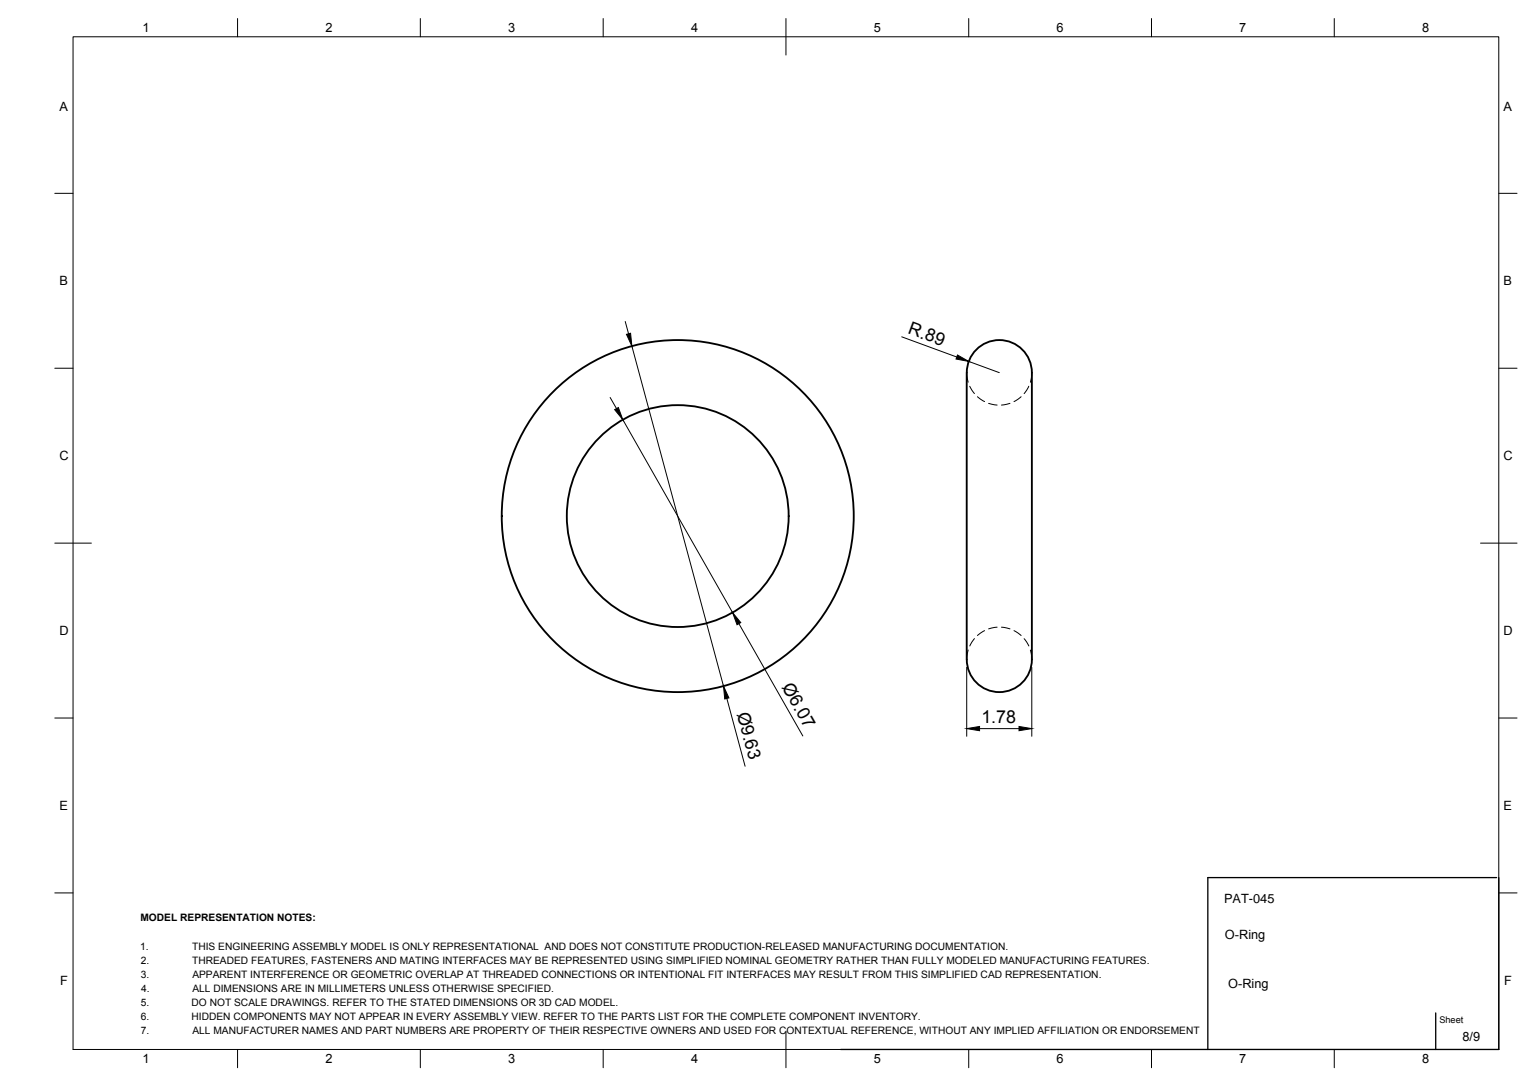
ISO-10303-21;
HEADER;
/* Generated by software containing ST-Developer
 * from STEP Tools, Inc. (www.steptools.com) 
 */

FILE_DESCRIPTION(
/* description */ ('Gauge isolation and snubber set'),
/* implementation_level */ '2;1');

FILE_NAME(
/* name */ 'O-Ring.step',
/* time_stamp */ '2026-10-29T16:58:15-07:00',
/* author */ (''),
/* organization */ (''),
/* preprocessor_version */ 'ST-DEVELOPER v20.2',
/* originating_system */ 'Autodesk Translation Framework v15.17.0.0',
/* authorisation */ '');

FILE_SCHEMA (('AUTOMOTIVE_DESIGN { 1 0 10303 214 3 1 1 }'));
ENDSEC;

DATA;
#10=MECHANICAL_DESIGN_GEOMETRIC_PRESENTATION_REPRESENTATION('',(#97),#4043);
#69=TOROIDAL_SURFACE('',#2504,0.3925,0.089);
#81=SHAPE_REPRESENTATION_RELATIONSHIP('SRR','None',#4088,#89);
#89=ADVANCED_BREP_SHAPE_REPRESENTATION('',(#107),#4040);
#97=STYLED_ITEM('',(#4204),#107);
#107=MANIFOLD_SOLID_BREP('Body1',#2214);
#337=FACE_OUTER_BOUND('',#500,.T.);
#500=EDGE_LOOP('',(#1943,#1944,#1945,#1946));
#622=CIRCLE('',#2505,0.089);
#623=CIRCLE('',#2506,0.3035);
#1136=VERTEX_POINT('',#3884);
#1410=EDGE_CURVE('',#1136,#1136,#622,.T.);
#1411=EDGE_CURVE('',#1136,#1136,#623,.T.);
#1943=ORIENTED_EDGE('',*,*,#1410,.F.);
#1944=ORIENTED_EDGE('',*,*,#1411,.T.);
#1945=ORIENTED_EDGE('',*,*,#1410,.T.);
#1946=ORIENTED_EDGE('',*,*,#1411,.F.);
#2181=ADVANCED_FACE('',(#337),#69,.T.);
#2214=CLOSED_SHELL('',(#2181));
#2503=AXIS2_PLACEMENT_3D('',#3882,#3087,#3088);
#2504=AXIS2_PLACEMENT_3D('',#3883,#3089,#3090);
#2505=AXIS2_PLACEMENT_3D('',#3885,#3091,#3092);
#2506=AXIS2_PLACEMENT_3D('',#3886,#3093,#3094);
#3087=DIRECTION('axis',(0.,0.,1.));
#3088=DIRECTION('refdir',(1.,0.,0.));
#3089=DIRECTION('center_axis',(0.,-1.,0.));
#3090=DIRECTION('ref_axis',(0.,0.,-1.));
#3091=DIRECTION('center_axis',(-1.,0.,-1.22464679914735E-16));
#3092=DIRECTION('ref_axis',(-1.22464679914735E-16,0.,1.));
#3093=DIRECTION('center_axis',(0.,1.,0.));
#3094=DIRECTION('ref_axis',(0.,0.,-1.));
#3882=CARTESIAN_POINT('',(0.,0.,0.));
#3883=CARTESIAN_POINT('Origin',(0.,0.,0.));
#3884=CARTESIAN_POINT('',(-3.71680303541222E-17,-1.08993565124114E-17,0.3035));
#3885=CARTESIAN_POINT('Origin',(-4.80673868665336E-17,0.,0.3925));
#3886=CARTESIAN_POINT('Origin',(0.,1.08993565124114E-17,0.));
#4029=UNCERTAINTY_MEASURE_WITH_UNIT(LENGTH_MEASURE(0.001),#4044,
'DISTANCE_ACCURACY_VALUE',
'Maximum model space distance between geometric entities at asserted c
onnectivities');
#4032=UNCERTAINTY_MEASURE_WITH_UNIT(LENGTH_MEASURE(0.001),#4044,
'DISTANCE_ACCURACY_VALUE',
'Maximum model space distance between geometric entities at asserted c
onnectivities');
#4040=(
GEOMETRIC_REPRESENTATION_CONTEXT(3)
GLOBAL_UNCERTAINTY_ASSIGNED_CONTEXT((#4029))
GLOBAL_UNIT_ASSIGNED_CONTEXT((#4044,#4046,#4047))
REPRESENTATION_CONTEXT('','3D')
);
#4043=(
GEOMETRIC_REPRESENTATION_CONTEXT(3)
GLOBAL_UNCERTAINTY_ASSIGNED_CONTEXT((#4032))
GLOBAL_UNIT_ASSIGNED_CONTEXT((#4044,#4046,#4047))
REPRESENTATION_CONTEXT('','3D')
);
#4044=(
LENGTH_UNIT()
NAMED_UNIT(*)
SI_UNIT(.CENTI.,.METRE.)
);
#4046=(
NAMED_UNIT(*)
PLANE_ANGLE_UNIT()
SI_UNIT($,.RADIAN.)
);
#4047=(
NAMED_UNIT(*)
SI_UNIT($,.STERADIAN.)
SOLID_ANGLE_UNIT()
);
#4055=SHAPE_DEFINITION_REPRESENTATION(#4065,#4088);
#4065=PRODUCT_DEFINITION_SHAPE('',$,#4099);
#4088=SHAPE_REPRESENTATION('',(#2503),#4040);
#4091=PRODUCT_DEFINITION_CONTEXT('part definition',#4123,'design');
#4099=PRODUCT_DEFINITION('O-Ring','O-Ring',#4109,#4091);
#4109=PRODUCT_DEFINITION_FORMATION('',$,#4132);
#4123=APPLICATION_CONTEXT(
'Core Data for Automotive Mechanical Design Process');
#4124=PRODUCT_CONTEXT('part definition',#4123,'mechanical');
#4132=PRODUCT('O-Ring','O-Ring','O-Ring',(#4124));
#4198=COLOUR_RGB('Black',0.12,0.14,0.17);
#4199=FILL_AREA_STYLE_COLOUR('',#4198);
#4200=FILL_AREA_STYLE('',(#4199));
#4201=SURFACE_STYLE_FILL_AREA(#4200);
#4202=SURFACE_SIDE_STYLE('',(#4201));
#4203=SURFACE_STYLE_USAGE(.BOTH.,#4202);
#4204=PRESENTATION_STYLE_ASSIGNMENT((#4203));
ENDSEC;
END-ISO-10303-21;
